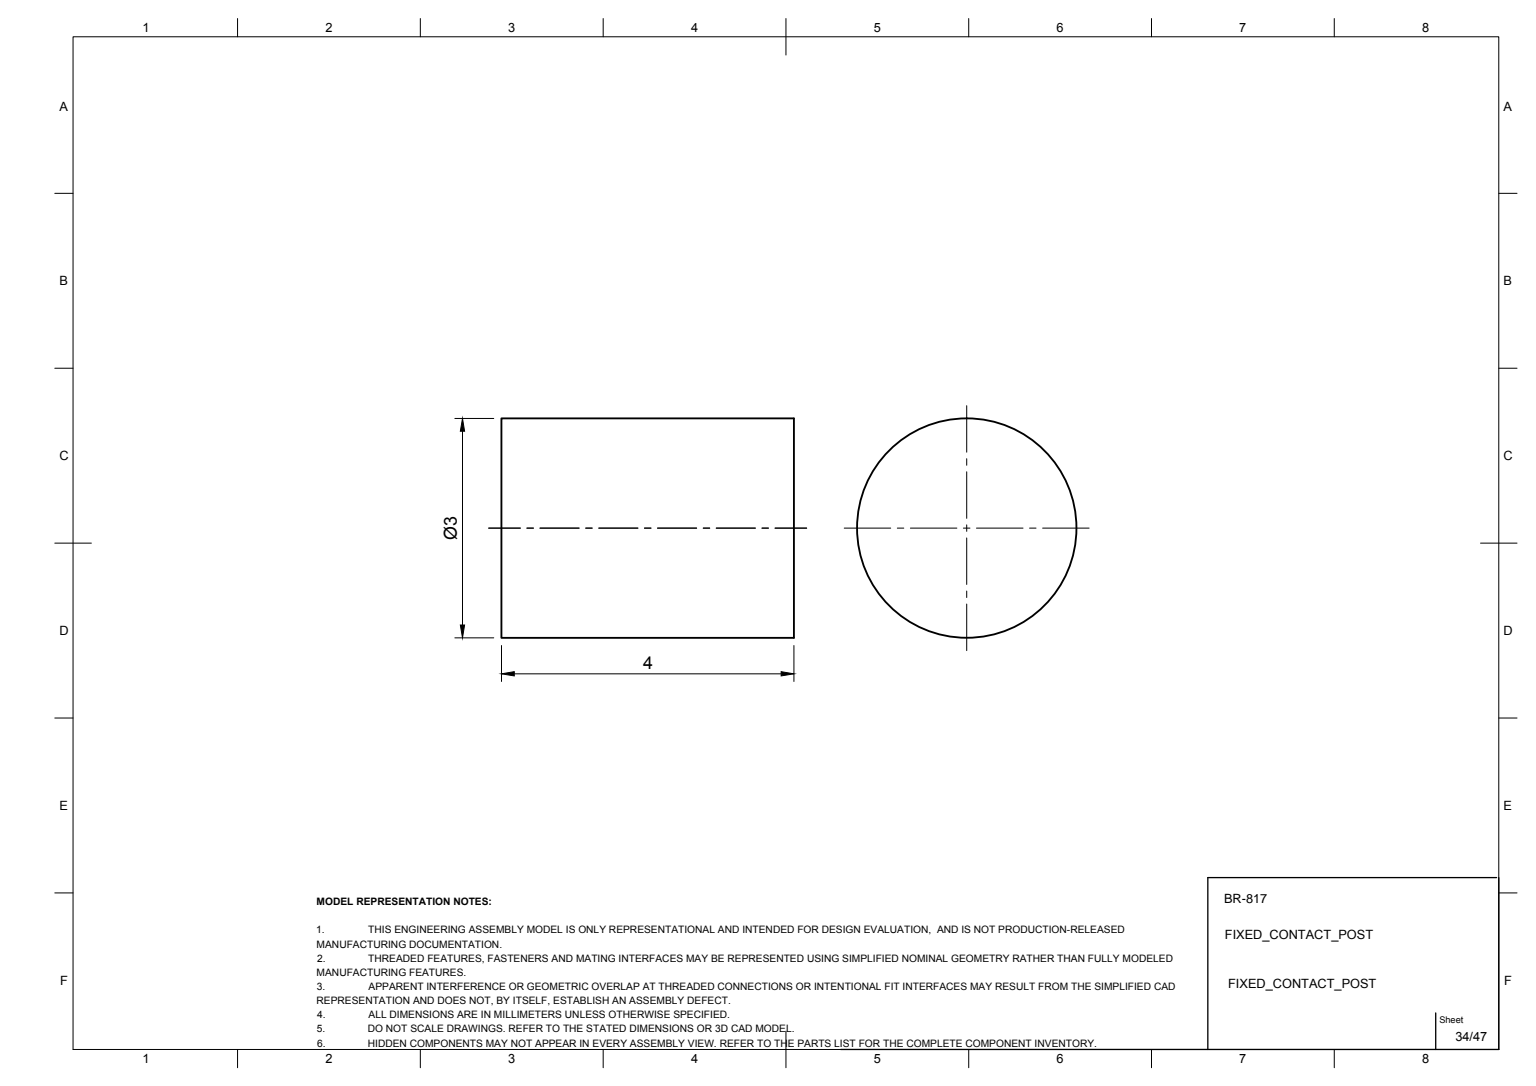
ISO-10303-21;
HEADER;
FILE_DESCRIPTION((''),'2;1');
FILE_NAME('FIXED_CONTACT_POST.step','2026-10-01T22:07:29-07:00',(''),(''),'','','');
FILE_SCHEMA (('AUTOMOTIVE_DESIGN { 1 0 10303 214 3 1 1 }'));
ENDSEC;
DATA;
#10=MECHANICAL_DESIGN_GEOMETRIC_PRESENTATION_REPRESENTATION('',(#567),#15484);
#496=SHAPE_REPRESENTATION_RELATIONSHIP('SRR','None',#15646,#531) ;
#531=ADVANCED_BREP_SHAPE_REPRESENTATION('',(#608),#15470) ;
#567=STYLED_ITEM('',(#15834),#608) ;
#608=MANIFOLD_SOLID_BREP('FIXED_CONTACT_POST',#8278) ;
#759=CYLINDRICAL_SURFACE('',#9537,0.15) ;
#1225=CIRCLE('',#9538,0.15) ;
#1226=CIRCLE('',#9539,0.15) ;
#1718=FACE_OUTER_BOUND('',#2284,.T.) ;
#1719=FACE_OUTER_BOUND('',#2285,.T.) ;
#1720=FACE_OUTER_BOUND('',#2286,.T.) ;
#2284=EDGE_LOOP('',(#6885,#6886,#6887,#6888)) ;
#2285=EDGE_LOOP('',(#6889)) ;
#2286=EDGE_LOOP('',(#6890)) ;
#2786=LINE('',#14671,#3260) ;
#3260=VECTOR('',#11985,0.15) ;
#3925=VERTEX_POINT('',#14668) ;
#3926=VERTEX_POINT('',#14670) ;
#4947=EDGE_CURVE('',#3925,#3925,#1225,.T.) ;
#4948=EDGE_CURVE('',#3925,#3926,#2786,.T.) ;
#4949=EDGE_CURVE('',#3926,#3926,#1226,.T.) ;
#6885=ORIENTED_EDGE('',*,*,#4947,.F.) ;
#6886=ORIENTED_EDGE('',*,*,#4948,.T.) ;
#6887=ORIENTED_EDGE('',*,*,#4949,.F.) ;
#6888=ORIENTED_EDGE('',*,*,#4948,.F.) ;
#6889=ORIENTED_EDGE('',*,*,#4949,.T.) ;
#6890=ORIENTED_EDGE('',*,*,#4947,.T.) ;
#7689=PLANE('',#9540) ;
#7690=PLANE('',#9541) ;
#8105=ADVANCED_FACE('',(#1718),#759,.T.) ;
#8106=ADVANCED_FACE('',(#1719),#7689,.T.) ;
#8107=ADVANCED_FACE('',(#1720),#7690,.T.) ;
#8278=CLOSED_SHELL('',(#8105,#8106,#8107)) ;
#9536=AXIS2_PLACEMENT_3D('',#14666,#11979,#11980) ;
#9537=AXIS2_PLACEMENT_3D('',#14667,#11981,#11982) ;
#9538=AXIS2_PLACEMENT_3D('',#14669,#11983,#11984) ;
#9539=AXIS2_PLACEMENT_3D('',#14672,#11986,#11987) ;
#9540=AXIS2_PLACEMENT_3D('',#14673,#11988,#11989) ;
#9541=AXIS2_PLACEMENT_3D('',#14674,#11990,#11991) ;
#11979=DIRECTION('axis',(0.,0.,1.)) ;
#11980=DIRECTION('refdir',(1.,0.,0.)) ;
#11981=DIRECTION('center_axis',(0.,0.,1.)) ;
#11982=DIRECTION('ref_axis',(1.,0.,0.)) ;
#11983=DIRECTION('center_axis',(0.,0.,1.)) ;
#11984=DIRECTION('ref_axis',(1.,0.,0.)) ;
#11985=DIRECTION('',(0.,0.,-1.)) ;
#11986=DIRECTION('center_axis',(0.,0.,-1.)) ;
#11987=DIRECTION('ref_axis',(1.,0.,0.)) ;
#11988=DIRECTION('center_axis',(0.,0.,-1.)) ;
#11989=DIRECTION('ref_axis',(-1.,0.,0.)) ;
#11990=DIRECTION('center_axis',(0.,0.,1.)) ;
#11991=DIRECTION('ref_axis',(1.,0.,0.)) ;
#14666=CARTESIAN_POINT('',(0.,0.,0.)) ;
#14667=CARTESIAN_POINT('Origin',(-1.1,-1.75,0.5)) ;
#14668=CARTESIAN_POINT('',(-1.25,-1.75,0.7)) ;
#14669=CARTESIAN_POINT('Origin',(-1.1,-1.75,0.7)) ;
#14670=CARTESIAN_POINT('',(-1.25,-1.75,0.3)) ;
#14671=CARTESIAN_POINT('',(-1.25,-1.75,0.5)) ;
#14672=CARTESIAN_POINT('Origin',(-1.1,-1.75,0.3)) ;
#14673=CARTESIAN_POINT('Origin',(-1.1,-1.75,0.3)) ;
#14674=CARTESIAN_POINT('Origin',(-1.1,-1.75,0.7)) ;
#15427=UNCERTAINTY_MEASURE_WITH_UNIT(LENGTH_MEASURE(0.001),#15485,
'DISTANCE_ACCURACY_VALUE',
'Maximum model space distance between geometric entities at asserted c
onnectivities') ;
#15441=UNCERTAINTY_MEASURE_WITH_UNIT(LENGTH_MEASURE(0.001),#15485,
'DISTANCE_ACCURACY_VALUE',
'Maximum model space distance between geometric entities at asserted c
onnectivities') ;
#15470=(
GEOMETRIC_REPRESENTATION_CONTEXT(3)
GLOBAL_UNCERTAINTY_ASSIGNED_CONTEXT((#15427))
GLOBAL_UNIT_ASSIGNED_CONTEXT((#15485,#15487,#15488))
REPRESENTATION_CONTEXT('','3D')
) ;
#15484=(
GEOMETRIC_REPRESENTATION_CONTEXT(3)
GLOBAL_UNCERTAINTY_ASSIGNED_CONTEXT((#15441))
GLOBAL_UNIT_ASSIGNED_CONTEXT((#15485,#15487,#15488))
REPRESENTATION_CONTEXT('','3D')
) ;
#15485=(
LENGTH_UNIT()
NAMED_UNIT(*)
SI_UNIT(.CENTI.,.METRE.)
) ;
#15487=(
NAMED_UNIT(*)
PLANE_ANGLE_UNIT()
SI_UNIT($,.RADIAN.)
) ;
#15488=(
NAMED_UNIT(*)
SI_UNIT($,.STERADIAN.)
SOLID_ANGLE_UNIT()
) ;
#15517=SHAPE_DEFINITION_REPRESENTATION(#15574,#15646) ;
#15574=PRODUCT_DEFINITION_SHAPE('',$,#15689) ;
#15646=SHAPE_REPRESENTATION('',(#9536),#15470) ;
#15660=PRODUCT_DEFINITION_CONTEXT('part definition',#15788,'design') ;
#15689=PRODUCT_DEFINITION('FIXED_CONTACT_POST',
'FIXED_CONTACT_POST',#15731,#15660) ;
#15731=PRODUCT_DEFINITION_FORMATION('',$,#15818) ;
#15788=APPLICATION_CONTEXT(
'Core Data for Automotive Mechanical Design Process') ;
#15789=PRODUCT_CONTEXT('part definition',#15788,'mechanical') ;
#15818=PRODUCT('FIXED_CONTACT_POST','FIXED_CONTACT_POST',$,(#15789)) ;
#15834=PRESENTATION_STYLE_ASSIGNMENT((#15846)) ;
#15846=SURFACE_STYLE_USAGE(.BOTH.,#15858) ;
#15858=SURFACE_SIDE_STYLE('',(#15870)) ;
#15870=SURFACE_STYLE_FILL_AREA(#15882) ;
#15882=FILL_AREA_STYLE('Brass - Polished',(#15894)) ;
#15894=FILL_AREA_STYLE_COLOUR('Brass - Polished',#15906) ;
#15906=COLOUR_RGB('Brass - Polished', 0.08235294, 0.09019608, 0.10196078) ;
ENDSEC;
END-ISO-10303-21;
